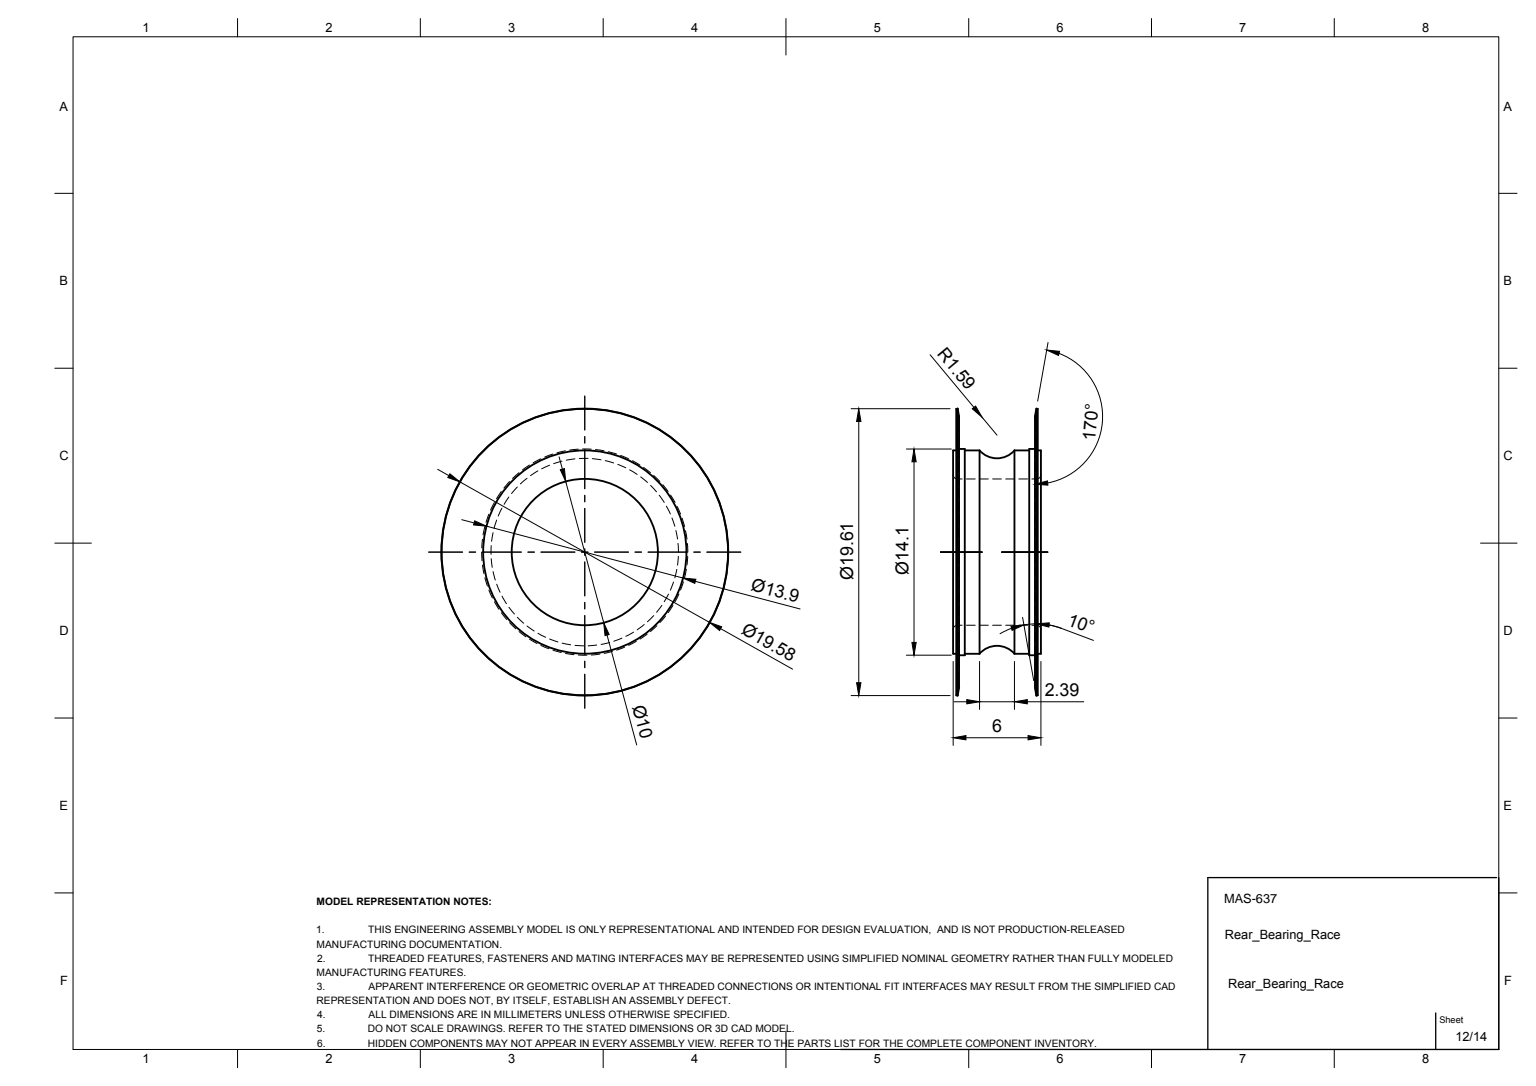
ISO-10303-21;
HEADER;
FILE_DESCRIPTION((''),'2;1');
FILE_NAME('Rear_Bearing_Race.step','2026-10-09T10:11:57-07:00',(''),(''),'','','');
FILE_SCHEMA (('AUTOMOTIVE_DESIGN { 1 0 10303 214 3 1 1 }'));
ENDSEC;
DATA;
#10=MECHANICAL_DESIGN_GEOMETRIC_PRESENTATION_REPRESENTATION('',(#144),#13510);
#105=SHAPE_REPRESENTATION_RELATIONSHIP('SRR','None',#13575,#120) ;
#120=ADVANCED_BREP_SHAPE_REPRESENTATION('',(#176),#13507) ;
#144=STYLED_ITEM('',(#13650),#176) ;
#176=MANIFOLD_SOLID_BREP('Body1',#7393) ;
#256=FACE_BOUND('',#1578,.T.) ;
#257=FACE_BOUND('',#1589,.T.) ;
#258=FACE_BOUND('',#1593,.T.) ;
#259=FACE_BOUND('',#1597,.T.) ;
#260=FACE_BOUND('',#1599,.T.) ;
#261=FACE_BOUND('',#1608,.T.) ;
#262=FACE_BOUND('',#1616,.T.) ;
#263=FACE_BOUND('',#1620,.T.) ;
#464=PLANE('',#8408) ;
#465=PLANE('',#8432) ;
#466=PLANE('',#8439) ;
#467=PLANE('',#8447) ;
#468=PLANE('',#8449) ;
#469=PLANE('',#8469) ;
#470=PLANE('',#8484) ;
#471=PLANE('',#8491) ;
#521=TOROIDAL_SURFACE('',#8404,7.1,0.15) ;
#522=TOROIDAL_SURFACE('',#8410,8.92946920772,0.45) ;
#523=TOROIDAL_SURFACE('',#8415,9.22752171828,0.349999999988) ;
#524=TOROIDAL_SURFACE('',#8424,9.22752171828,0.45) ;
#525=TOROIDAL_SURFACE('',#8429,8.92946920772,0.35) ;
#526=TOROIDAL_SURFACE('',#8434,7.1,0.05) ;
#527=TOROIDAL_SURFACE('',#8441,7.1,0.15) ;
#528=TOROIDAL_SURFACE('',#8451,8.92946920772,0.45) ;
#529=TOROIDAL_SURFACE('',#8454,5.3,0.3) ;
#530=TOROIDAL_SURFACE('',#8461,9.22752171828,0.349999999988) ;
#531=TOROIDAL_SURFACE('',#8464,5.3,0.3) ;
#532=TOROIDAL_SURFACE('',#8476,9.22752171828,0.45) ;
#533=TOROIDAL_SURFACE('',#8481,8.92946920772,0.35) ;
#534=TOROIDAL_SURFACE('',#8486,7.1,0.05) ;
#535=TOROIDAL_SURFACE('',#8495,8.,1.59) ;
#656=CYLINDRICAL_SURFACE('',#8437,7.05) ;
#657=CYLINDRICAL_SURFACE('',#8445,6.95) ;
#658=CYLINDRICAL_SURFACE('',#8459,5.) ;
#659=CYLINDRICAL_SURFACE('',#8473,6.95) ;
#660=CYLINDRICAL_SURFACE('',#8489,7.05) ;
#661=CYLINDRICAL_SURFACE('',#8493,6.95) ;
#662=CYLINDRICAL_SURFACE('',#8498,6.95) ;
#1059=FACE_OUTER_BOUND('',#1576,.T.) ;
#1060=FACE_OUTER_BOUND('',#1577,.T.) ;
#1061=FACE_OUTER_BOUND('',#1579,.T.) ;
#1062=FACE_OUTER_BOUND('',#1580,.T.) ;
#1063=FACE_OUTER_BOUND('',#1581,.T.) ;
#1064=FACE_OUTER_BOUND('',#1582,.T.) ;
#1065=FACE_OUTER_BOUND('',#1583,.T.) ;
#1066=FACE_OUTER_BOUND('',#1584,.T.) ;
#1067=FACE_OUTER_BOUND('',#1585,.T.) ;
#1068=FACE_OUTER_BOUND('',#1586,.T.) ;
#1069=FACE_OUTER_BOUND('',#1587,.T.) ;
#1070=FACE_OUTER_BOUND('',#1588,.T.) ;
#1071=FACE_OUTER_BOUND('',#1590,.T.) ;
#1072=FACE_OUTER_BOUND('',#1591,.T.) ;
#1073=FACE_OUTER_BOUND('',#1592,.T.) ;
#1074=FACE_OUTER_BOUND('',#1594,.T.) ;
#1075=FACE_OUTER_BOUND('',#1595,.T.) ;
#1076=FACE_OUTER_BOUND('',#1596,.T.) ;
#1077=FACE_OUTER_BOUND('',#1598,.T.) ;
#1078=FACE_OUTER_BOUND('',#1600,.T.) ;
#1079=FACE_OUTER_BOUND('',#1601,.T.) ;
#1080=FACE_OUTER_BOUND('',#1602,.T.) ;
#1081=FACE_OUTER_BOUND('',#1603,.T.) ;
#1082=FACE_OUTER_BOUND('',#1604,.T.) ;
#1083=FACE_OUTER_BOUND('',#1605,.T.) ;
#1084=FACE_OUTER_BOUND('',#1606,.T.) ;
#1085=FACE_OUTER_BOUND('',#1607,.T.) ;
#1086=FACE_OUTER_BOUND('',#1609,.T.) ;
#1087=FACE_OUTER_BOUND('',#1610,.T.) ;
#1088=FACE_OUTER_BOUND('',#1611,.T.) ;
#1089=FACE_OUTER_BOUND('',#1612,.T.) ;
#1090=FACE_OUTER_BOUND('',#1613,.T.) ;
#1091=FACE_OUTER_BOUND('',#1614,.T.) ;
#1092=FACE_OUTER_BOUND('',#1615,.T.) ;
#1093=FACE_OUTER_BOUND('',#1617,.T.) ;
#1094=FACE_OUTER_BOUND('',#1618,.T.) ;
#1095=FACE_OUTER_BOUND('',#1619,.T.) ;
#1096=FACE_OUTER_BOUND('',#1621,.T.) ;
#1097=FACE_OUTER_BOUND('',#1622,.T.) ;
#1098=FACE_OUTER_BOUND('',#1623,.T.) ;
#1576=EDGE_LOOP('',(#6656,#6657,#6658,#6659)) ;
#1577=EDGE_LOOP('',(#6660)) ;
#1578=EDGE_LOOP('',(#6661)) ;
#1579=EDGE_LOOP('',(#6662,#6663,#6664,#6665)) ;
#1580=EDGE_LOOP('',(#6666,#6667,#6668,#6669)) ;
#1581=EDGE_LOOP('',(#6670,#6671,#6672,#6673)) ;
#1582=EDGE_LOOP('',(#6674,#6675,#6676,#6677)) ;
#1583=EDGE_LOOP('',(#6678,#6679,#6680,#6681)) ;
#1584=EDGE_LOOP('',(#6682,#6683,#6684,#6685)) ;
#1585=EDGE_LOOP('',(#6686,#6687,#6688,#6689)) ;
#1586=EDGE_LOOP('',(#6690,#6691,#6692,#6693)) ;
#1587=EDGE_LOOP('',(#6694,#6695,#6696,#6697)) ;
#1588=EDGE_LOOP('',(#6698)) ;
#1589=EDGE_LOOP('',(#6699)) ;
#1590=EDGE_LOOP('',(#6700,#6701,#6702,#6703)) ;
#1591=EDGE_LOOP('',(#6704,#6705,#6706,#6707)) ;
#1592=EDGE_LOOP('',(#6708)) ;
#1593=EDGE_LOOP('',(#6709)) ;
#1594=EDGE_LOOP('',(#6710,#6711,#6712,#6713)) ;
#1595=EDGE_LOOP('',(#6714,#6715,#6716,#6717)) ;
#1596=EDGE_LOOP('',(#6718)) ;
#1597=EDGE_LOOP('',(#6719)) ;
#1598=EDGE_LOOP('',(#6720)) ;
#1599=EDGE_LOOP('',(#6721)) ;
#1600=EDGE_LOOP('',(#6722,#6723,#6724,#6725)) ;
#1601=EDGE_LOOP('',(#6726,#6727,#6728,#6729)) ;
#1602=EDGE_LOOP('',(#6730,#6731,#6732,#6733)) ;
#1603=EDGE_LOOP('',(#6734,#6735,#6736,#6737)) ;
#1604=EDGE_LOOP('',(#6738,#6739,#6740,#6741)) ;
#1605=EDGE_LOOP('',(#6742,#6743,#6744,#6745)) ;
#1606=EDGE_LOOP('',(#6746,#6747,#6748,#6749)) ;
#1607=EDGE_LOOP('',(#6750)) ;
#1608=EDGE_LOOP('',(#6751)) ;
#1609=EDGE_LOOP('',(#6752,#6753,#6754,#6755)) ;
#1610=EDGE_LOOP('',(#6756,#6757,#6758,#6759)) ;
#1611=EDGE_LOOP('',(#6760,#6761,#6762,#6763)) ;
#1612=EDGE_LOOP('',(#6764,#6765,#6766,#6767)) ;
#1613=EDGE_LOOP('',(#6768,#6769,#6770,#6771)) ;
#1614=EDGE_LOOP('',(#6772,#6773,#6774,#6775)) ;
#1615=EDGE_LOOP('',(#6776)) ;
#1616=EDGE_LOOP('',(#6777)) ;
#1617=EDGE_LOOP('',(#6778,#6779,#6780,#6781)) ;
#1618=EDGE_LOOP('',(#6782,#6783,#6784,#6785)) ;
#1619=EDGE_LOOP('',(#6786)) ;
#1620=EDGE_LOOP('',(#6787)) ;
#1621=EDGE_LOOP('',(#6788,#6789,#6790,#6791)) ;
#1622=EDGE_LOOP('',(#6792,#6793,#6794,#6795)) ;
#1623=EDGE_LOOP('',(#6796,#6797,#6798,#6799)) ;
#2119=LINE('',#13234,#2613) ;
#2120=LINE('',#13241,#2614) ;
#2121=LINE('',#13246,#2615) ;
#2122=LINE('',#13249,#2616) ;
#2123=LINE('',#13258,#2617) ;
#2124=LINE('',#13272,#2618) ;
#2125=LINE('',#13285,#2619) ;
#2126=LINE('',#13304,#2620) ;
#2127=LINE('',#13307,#2621) ;
#2128=LINE('',#13319,#2622) ;
#2129=LINE('',#13327,#2623) ;
#2130=LINE('',#13329,#2624) ;
#2131=LINE('',#13332,#2625) ;
#2132=LINE('',#13341,#2626) ;
#2133=LINE('',#13356,#2627) ;
#2134=LINE('',#13363,#2628) ;
#2135=LINE('',#13369,#2629) ;
#2613=VECTOR('',#10727,9.08337827221) ;
#2614=VECTOR('',#10736,9.28829858046) ;
#2615=VECTOR('',#10743,9.78979836642) ;
#2616=VECTOR('',#10746,9.30566339823) ;
#2617=VECTOR('',#10759,9.04917625788) ;
#2618=VECTOR('',#10778,7.05) ;
#2619=VECTOR('',#10795,6.95) ;
#2620=VECTOR('',#10822,9.08337827221) ;
#2621=VECTOR('',#10825,5.) ;
#2622=VECTOR('',#10842,9.28829858046) ;
#2623=VECTOR('',#10853,9.78979836642) ;
#2624=VECTOR('',#10856,6.95) ;
#2625=VECTOR('',#10859,9.30566339823) ;
#2626=VECTOR('',#10872,9.04917625788) ;
#2627=VECTOR('',#10893,7.05) ;
#2628=VECTOR('',#10902,6.95) ;
#2629=VECTOR('',#10911,6.95) ;
#3060=CIRCLE('',#8405,6.95) ;
#3061=CIRCLE('',#8406,0.15) ;
#3062=CIRCLE('',#8407,7.1) ;
#3063=CIRCLE('',#8409,8.92946920772) ;
#3064=CIRCLE('',#8411,0.45) ;
#3065=CIRCLE('',#8412,9.08337827221) ;
#3066=CIRCLE('',#8414,9.10781466811) ;
#3067=CIRCLE('',#8416,0.349999999988) ;
#3068=CIRCLE('',#8417,9.28829858046) ;
#3069=CIRCLE('',#8419,9.78979836642) ;
#3070=CIRCLE('',#8421,9.80716318419) ;
#3071=CIRCLE('',#8423,9.30566339823) ;
#3072=CIRCLE('',#8425,0.45) ;
#3073=CIRCLE('',#8426,9.07361265378) ;
#3074=CIRCLE('',#8428,9.04917625788) ;
#3075=CIRCLE('',#8430,0.35) ;
#3076=CIRCLE('',#8431,8.92946920772) ;
#3077=CIRCLE('',#8433,7.1) ;
#3078=CIRCLE('',#8435,0.05) ;
#3079=CIRCLE('',#8436,7.05) ;
#3080=CIRCLE('',#8438,7.05) ;
#3081=CIRCLE('',#8440,6.95) ;
#3082=CIRCLE('',#8442,7.1) ;
#3083=CIRCLE('',#8443,0.15) ;
#3084=CIRCLE('',#8444,6.95) ;
#3085=CIRCLE('',#8446,6.95) ;
#3086=CIRCLE('',#8448,8.92946920772) ;
#3087=CIRCLE('',#8450,5.3) ;
#3088=CIRCLE('',#8452,9.08337827221) ;
#3089=CIRCLE('',#8453,0.45) ;
#3090=CIRCLE('',#8455,0.3) ;
#3091=CIRCLE('',#8456,5.) ;
#3092=CIRCLE('',#8458,9.10781466811) ;
#3093=CIRCLE('',#8460,5.) ;
#3094=CIRCLE('',#8462,9.28829858046) ;
#3095=CIRCLE('',#8463,0.349999999988) ;
#3096=CIRCLE('',#8465,0.3) ;
#3097=CIRCLE('',#8466,5.3) ;
#3098=CIRCLE('',#8468,9.78979836642) ;
#3099=CIRCLE('',#8470,6.95) ;
#3100=CIRCLE('',#8472,9.80716318419) ;
#3101=CIRCLE('',#8475,9.30566339823) ;
#3102=CIRCLE('',#8477,9.07361265378) ;
#3103=CIRCLE('',#8478,0.45) ;
#3104=CIRCLE('',#8480,9.04917625788) ;
#3105=CIRCLE('',#8482,8.92946920772) ;
#3106=CIRCLE('',#8483,0.35) ;
#3107=CIRCLE('',#8485,7.1) ;
#3108=CIRCLE('',#8487,7.05) ;
#3109=CIRCLE('',#8488,0.05) ;
#3110=CIRCLE('',#8490,7.05) ;
#3111=CIRCLE('',#8492,6.95) ;
#3112=CIRCLE('',#8494,6.95) ;
#3113=CIRCLE('',#8496,6.95) ;
#3114=CIRCLE('',#8497,1.59) ;
#3726=VERTEX_POINT('',#13219) ;
#3727=VERTEX_POINT('',#13221) ;
#3728=VERTEX_POINT('',#13225) ;
#3729=VERTEX_POINT('',#13228) ;
#3730=VERTEX_POINT('',#13232) ;
#3731=VERTEX_POINT('',#13236) ;
#3732=VERTEX_POINT('',#13240) ;
#3733=VERTEX_POINT('',#13244) ;
#3734=VERTEX_POINT('',#13248) ;
#3735=VERTEX_POINT('',#13252) ;
#3736=VERTEX_POINT('',#13256) ;
#3737=VERTEX_POINT('',#13260) ;
#3738=VERTEX_POINT('',#13264) ;
#3739=VERTEX_POINT('',#13267) ;
#3740=VERTEX_POINT('',#13271) ;
#3741=VERTEX_POINT('',#13275) ;
#3742=VERTEX_POINT('',#13278) ;
#3743=VERTEX_POINT('',#13280) ;
#3744=VERTEX_POINT('',#13284) ;
#3745=VERTEX_POINT('',#13288) ;
#3746=VERTEX_POINT('',#13291) ;
#3747=VERTEX_POINT('',#13294) ;
#3748=VERTEX_POINT('',#13298) ;
#3749=VERTEX_POINT('',#13302) ;
#3750=VERTEX_POINT('',#13306) ;
#3751=VERTEX_POINT('',#13310) ;
#3752=VERTEX_POINT('',#13314) ;
#3753=VERTEX_POINT('',#13318) ;
#3754=VERTEX_POINT('',#13322) ;
#3755=VERTEX_POINT('',#13325) ;
#3756=VERTEX_POINT('',#13331) ;
#3757=VERTEX_POINT('',#13335) ;
#3758=VERTEX_POINT('',#13339) ;
#3759=VERTEX_POINT('',#13343) ;
#3760=VERTEX_POINT('',#13347) ;
#3761=VERTEX_POINT('',#13350) ;
#3762=VERTEX_POINT('',#13354) ;
#3763=VERTEX_POINT('',#13358) ;
#3764=VERTEX_POINT('',#13361) ;
#3765=VERTEX_POINT('',#13365) ;
#4715=EDGE_CURVE('',#3726,#3726,#3060,.T.) ;
#4716=EDGE_CURVE('',#3726,#3727,#3061,.T.) ;
#4717=EDGE_CURVE('',#3727,#3727,#3062,.T.) ;
#4718=EDGE_CURVE('',#3728,#3728,#3063,.T.) ;
#4719=EDGE_CURVE('',#3728,#3729,#3064,.T.) ;
#4720=EDGE_CURVE('',#3729,#3729,#3065,.T.) ;
#4721=EDGE_CURVE('',#3730,#3730,#3066,.F.) ;
#4722=EDGE_CURVE('',#3730,#3729,#2119,.T.) ;
#4723=EDGE_CURVE('',#3730,#3731,#3067,.T.) ;
#4724=EDGE_CURVE('',#3731,#3731,#3068,.T.) ;
#4725=EDGE_CURVE('',#3731,#3732,#2120,.T.) ;
#4726=EDGE_CURVE('',#3732,#3732,#3069,.T.) ;
#4727=EDGE_CURVE('',#3733,#3733,#3070,.F.) ;
#4728=EDGE_CURVE('',#3733,#3732,#2121,.T.) ;
#4729=EDGE_CURVE('',#3733,#3734,#2122,.T.) ;
#4730=EDGE_CURVE('',#3734,#3734,#3071,.T.) ;
#4731=EDGE_CURVE('',#3734,#3735,#3072,.T.) ;
#4732=EDGE_CURVE('',#3735,#3735,#3073,.T.) ;
#4733=EDGE_CURVE('',#3736,#3736,#3074,.F.) ;
#4734=EDGE_CURVE('',#3736,#3735,#2123,.T.) ;
#4735=EDGE_CURVE('',#3736,#3737,#3075,.T.) ;
#4736=EDGE_CURVE('',#3737,#3737,#3076,.T.) ;
#4737=EDGE_CURVE('',#3738,#3738,#3077,.T.) ;
#4738=EDGE_CURVE('',#3738,#3739,#3078,.T.) ;
#4739=EDGE_CURVE('',#3739,#3739,#3079,.T.) ;
#4740=EDGE_CURVE('',#3739,#3740,#2124,.T.) ;
#4741=EDGE_CURVE('',#3740,#3740,#3080,.T.) ;
#4742=EDGE_CURVE('',#3741,#3741,#3081,.T.) ;
#4743=EDGE_CURVE('',#3742,#3742,#3082,.T.) ;
#4744=EDGE_CURVE('',#3742,#3743,#3083,.T.) ;
#4745=EDGE_CURVE('',#3743,#3743,#3084,.T.) ;
#4746=EDGE_CURVE('',#3743,#3744,#2125,.T.) ;
#4747=EDGE_CURVE('',#3744,#3744,#3085,.T.) ;
#4748=EDGE_CURVE('',#3745,#3745,#3086,.T.) ;
#4749=EDGE_CURVE('',#3746,#3746,#3087,.T.) ;
#4750=EDGE_CURVE('',#3747,#3747,#3088,.T.) ;
#4751=EDGE_CURVE('',#3747,#3745,#3089,.T.) ;
#4752=EDGE_CURVE('',#3746,#3748,#3090,.T.) ;
#4753=EDGE_CURVE('',#3748,#3748,#3091,.T.) ;
#4754=EDGE_CURVE('',#3749,#3749,#3092,.T.) ;
#4755=EDGE_CURVE('',#3749,#3747,#2126,.T.) ;
#4756=EDGE_CURVE('',#3748,#3750,#2127,.T.) ;
#4757=EDGE_CURVE('',#3750,#3750,#3093,.T.) ;
#4758=EDGE_CURVE('',#3751,#3751,#3094,.T.) ;
#4759=EDGE_CURVE('',#3751,#3749,#3095,.T.) ;
#4760=EDGE_CURVE('',#3750,#3752,#3096,.T.) ;
#4761=EDGE_CURVE('',#3752,#3752,#3097,.T.) ;
#4762=EDGE_CURVE('',#3751,#3753,#2128,.T.) ;
#4763=EDGE_CURVE('',#3753,#3753,#3098,.F.) ;
#4764=EDGE_CURVE('',#3754,#3754,#3099,.T.) ;
#4765=EDGE_CURVE('',#3755,#3755,#3100,.T.) ;
#4766=EDGE_CURVE('',#3755,#3753,#2129,.T.) ;
#4767=EDGE_CURVE('',#3754,#3726,#2130,.T.) ;
#4768=EDGE_CURVE('',#3755,#3756,#2131,.T.) ;
#4769=EDGE_CURVE('',#3756,#3756,#3101,.F.) ;
#4770=EDGE_CURVE('',#3757,#3757,#3102,.T.) ;
#4771=EDGE_CURVE('',#3757,#3756,#3103,.T.) ;
#4772=EDGE_CURVE('',#3758,#3758,#3104,.T.) ;
#4773=EDGE_CURVE('',#3758,#3757,#2132,.T.) ;
#4774=EDGE_CURVE('',#3759,#3759,#3105,.T.) ;
#4775=EDGE_CURVE('',#3759,#3758,#3106,.T.) ;
#4776=EDGE_CURVE('',#3760,#3760,#3107,.T.) ;
#4777=EDGE_CURVE('',#3761,#3761,#3108,.T.) ;
#4778=EDGE_CURVE('',#3761,#3760,#3109,.T.) ;
#4779=EDGE_CURVE('',#3762,#3762,#3110,.T.) ;
#4780=EDGE_CURVE('',#3762,#3761,#2133,.T.) ;
#4781=EDGE_CURVE('',#3763,#3763,#3111,.T.) ;
#4782=EDGE_CURVE('',#3764,#3764,#3112,.T.) ;
#4783=EDGE_CURVE('',#3764,#3763,#2134,.T.) ;
#4784=EDGE_CURVE('',#3765,#3765,#3113,.T.) ;
#4785=EDGE_CURVE('',#3765,#3764,#3114,.T.) ;
#4786=EDGE_CURVE('',#3741,#3765,#2135,.T.) ;
#6656=ORIENTED_EDGE('',*,*,#4715,.F.) ;
#6657=ORIENTED_EDGE('',*,*,#4716,.T.) ;
#6658=ORIENTED_EDGE('',*,*,#4717,.T.) ;
#6659=ORIENTED_EDGE('',*,*,#4716,.F.) ;
#6660=ORIENTED_EDGE('',*,*,#4718,.T.) ;
#6661=ORIENTED_EDGE('',*,*,#4717,.F.) ;
#6662=ORIENTED_EDGE('',*,*,#4718,.F.) ;
#6663=ORIENTED_EDGE('',*,*,#4719,.T.) ;
#6664=ORIENTED_EDGE('',*,*,#4720,.T.) ;
#6665=ORIENTED_EDGE('',*,*,#4719,.F.) ;
#6666=ORIENTED_EDGE('',*,*,#4721,.T.) ;
#6667=ORIENTED_EDGE('',*,*,#4722,.T.) ;
#6668=ORIENTED_EDGE('',*,*,#4720,.F.) ;
#6669=ORIENTED_EDGE('',*,*,#4722,.F.) ;
#6670=ORIENTED_EDGE('',*,*,#4721,.F.) ;
#6671=ORIENTED_EDGE('',*,*,#4723,.T.) ;
#6672=ORIENTED_EDGE('',*,*,#4724,.T.) ;
#6673=ORIENTED_EDGE('',*,*,#4723,.F.) ;
#6674=ORIENTED_EDGE('',*,*,#4724,.F.) ;
#6675=ORIENTED_EDGE('',*,*,#4725,.T.) ;
#6676=ORIENTED_EDGE('',*,*,#4726,.T.) ;
#6677=ORIENTED_EDGE('',*,*,#4725,.F.) ;
#6678=ORIENTED_EDGE('',*,*,#4727,.T.) ;
#6679=ORIENTED_EDGE('',*,*,#4728,.T.) ;
#6680=ORIENTED_EDGE('',*,*,#4726,.F.) ;
#6681=ORIENTED_EDGE('',*,*,#4728,.F.) ;
#6682=ORIENTED_EDGE('',*,*,#4727,.F.) ;
#6683=ORIENTED_EDGE('',*,*,#4729,.T.) ;
#6684=ORIENTED_EDGE('',*,*,#4730,.T.) ;
#6685=ORIENTED_EDGE('',*,*,#4729,.F.) ;
#6686=ORIENTED_EDGE('',*,*,#4730,.F.) ;
#6687=ORIENTED_EDGE('',*,*,#4731,.T.) ;
#6688=ORIENTED_EDGE('',*,*,#4732,.T.) ;
#6689=ORIENTED_EDGE('',*,*,#4731,.F.) ;
#6690=ORIENTED_EDGE('',*,*,#4733,.T.) ;
#6691=ORIENTED_EDGE('',*,*,#4734,.T.) ;
#6692=ORIENTED_EDGE('',*,*,#4732,.F.) ;
#6693=ORIENTED_EDGE('',*,*,#4734,.F.) ;
#6694=ORIENTED_EDGE('',*,*,#4733,.F.) ;
#6695=ORIENTED_EDGE('',*,*,#4735,.T.) ;
#6696=ORIENTED_EDGE('',*,*,#4736,.T.) ;
#6697=ORIENTED_EDGE('',*,*,#4735,.F.) ;
#6698=ORIENTED_EDGE('',*,*,#4736,.F.) ;
#6699=ORIENTED_EDGE('',*,*,#4737,.T.) ;
#6700=ORIENTED_EDGE('',*,*,#4737,.F.) ;
#6701=ORIENTED_EDGE('',*,*,#4738,.T.) ;
#6702=ORIENTED_EDGE('',*,*,#4739,.T.) ;
#6703=ORIENTED_EDGE('',*,*,#4738,.F.) ;
#6704=ORIENTED_EDGE('',*,*,#4739,.F.) ;
#6705=ORIENTED_EDGE('',*,*,#4740,.T.) ;
#6706=ORIENTED_EDGE('',*,*,#4741,.T.) ;
#6707=ORIENTED_EDGE('',*,*,#4740,.F.) ;
#6708=ORIENTED_EDGE('',*,*,#4741,.F.) ;
#6709=ORIENTED_EDGE('',*,*,#4742,.T.) ;
#6710=ORIENTED_EDGE('',*,*,#4743,.F.) ;
#6711=ORIENTED_EDGE('',*,*,#4744,.T.) ;
#6712=ORIENTED_EDGE('',*,*,#4745,.T.) ;
#6713=ORIENTED_EDGE('',*,*,#4744,.F.) ;
#6714=ORIENTED_EDGE('',*,*,#4745,.F.) ;
#6715=ORIENTED_EDGE('',*,*,#4746,.T.) ;
#6716=ORIENTED_EDGE('',*,*,#4747,.T.) ;
#6717=ORIENTED_EDGE('',*,*,#4746,.F.) ;
#6718=ORIENTED_EDGE('',*,*,#4748,.F.) ;
#6719=ORIENTED_EDGE('',*,*,#4743,.T.) ;
#6720=ORIENTED_EDGE('',*,*,#4747,.F.) ;
#6721=ORIENTED_EDGE('',*,*,#4749,.T.) ;
#6722=ORIENTED_EDGE('',*,*,#4750,.F.) ;
#6723=ORIENTED_EDGE('',*,*,#4751,.T.) ;
#6724=ORIENTED_EDGE('',*,*,#4748,.T.) ;
#6725=ORIENTED_EDGE('',*,*,#4751,.F.) ;
#6726=ORIENTED_EDGE('',*,*,#4749,.F.) ;
#6727=ORIENTED_EDGE('',*,*,#4752,.T.) ;
#6728=ORIENTED_EDGE('',*,*,#4753,.T.) ;
#6729=ORIENTED_EDGE('',*,*,#4752,.F.) ;
#6730=ORIENTED_EDGE('',*,*,#4754,.F.) ;
#6731=ORIENTED_EDGE('',*,*,#4755,.T.) ;
#6732=ORIENTED_EDGE('',*,*,#4750,.T.) ;
#6733=ORIENTED_EDGE('',*,*,#4755,.F.) ;
#6734=ORIENTED_EDGE('',*,*,#4753,.F.) ;
#6735=ORIENTED_EDGE('',*,*,#4756,.T.) ;
#6736=ORIENTED_EDGE('',*,*,#4757,.T.) ;
#6737=ORIENTED_EDGE('',*,*,#4756,.F.) ;
#6738=ORIENTED_EDGE('',*,*,#4758,.F.) ;
#6739=ORIENTED_EDGE('',*,*,#4759,.T.) ;
#6740=ORIENTED_EDGE('',*,*,#4754,.T.) ;
#6741=ORIENTED_EDGE('',*,*,#4759,.F.) ;
#6742=ORIENTED_EDGE('',*,*,#4757,.F.) ;
#6743=ORIENTED_EDGE('',*,*,#4760,.T.) ;
#6744=ORIENTED_EDGE('',*,*,#4761,.T.) ;
#6745=ORIENTED_EDGE('',*,*,#4760,.F.) ;
#6746=ORIENTED_EDGE('',*,*,#4758,.T.) ;
#6747=ORIENTED_EDGE('',*,*,#4762,.T.) ;
#6748=ORIENTED_EDGE('',*,*,#4763,.F.) ;
#6749=ORIENTED_EDGE('',*,*,#4762,.F.) ;
#6750=ORIENTED_EDGE('',*,*,#4764,.T.) ;
#6751=ORIENTED_EDGE('',*,*,#4761,.F.) ;
#6752=ORIENTED_EDGE('',*,*,#4765,.F.) ;
#6753=ORIENTED_EDGE('',*,*,#4766,.T.) ;
#6754=ORIENTED_EDGE('',*,*,#4763,.T.) ;
#6755=ORIENTED_EDGE('',*,*,#4766,.F.) ;
#6756=ORIENTED_EDGE('',*,*,#4764,.F.) ;
#6757=ORIENTED_EDGE('',*,*,#4767,.T.) ;
#6758=ORIENTED_EDGE('',*,*,#4715,.T.) ;
#6759=ORIENTED_EDGE('',*,*,#4767,.F.) ;
#6760=ORIENTED_EDGE('',*,*,#4765,.T.) ;
#6761=ORIENTED_EDGE('',*,*,#4768,.T.) ;
#6762=ORIENTED_EDGE('',*,*,#4769,.F.) ;
#6763=ORIENTED_EDGE('',*,*,#4768,.F.) ;
#6764=ORIENTED_EDGE('',*,*,#4770,.F.) ;
#6765=ORIENTED_EDGE('',*,*,#4771,.T.) ;
#6766=ORIENTED_EDGE('',*,*,#4769,.T.) ;
#6767=ORIENTED_EDGE('',*,*,#4771,.F.) ;
#6768=ORIENTED_EDGE('',*,*,#4772,.F.) ;
#6769=ORIENTED_EDGE('',*,*,#4773,.T.) ;
#6770=ORIENTED_EDGE('',*,*,#4770,.T.) ;
#6771=ORIENTED_EDGE('',*,*,#4773,.F.) ;
#6772=ORIENTED_EDGE('',*,*,#4774,.F.) ;
#6773=ORIENTED_EDGE('',*,*,#4775,.T.) ;
#6774=ORIENTED_EDGE('',*,*,#4772,.T.) ;
#6775=ORIENTED_EDGE('',*,*,#4775,.F.) ;
#6776=ORIENTED_EDGE('',*,*,#4774,.T.) ;
#6777=ORIENTED_EDGE('',*,*,#4776,.F.) ;
#6778=ORIENTED_EDGE('',*,*,#4777,.F.) ;
#6779=ORIENTED_EDGE('',*,*,#4778,.T.) ;
#6780=ORIENTED_EDGE('',*,*,#4776,.T.) ;
#6781=ORIENTED_EDGE('',*,*,#4778,.F.) ;
#6782=ORIENTED_EDGE('',*,*,#4779,.F.) ;
#6783=ORIENTED_EDGE('',*,*,#4780,.T.) ;
#6784=ORIENTED_EDGE('',*,*,#4777,.T.) ;
#6785=ORIENTED_EDGE('',*,*,#4780,.F.) ;
#6786=ORIENTED_EDGE('',*,*,#4779,.T.) ;
#6787=ORIENTED_EDGE('',*,*,#4781,.F.) ;
#6788=ORIENTED_EDGE('',*,*,#4782,.F.) ;
#6789=ORIENTED_EDGE('',*,*,#4783,.T.) ;
#6790=ORIENTED_EDGE('',*,*,#4781,.T.) ;
#6791=ORIENTED_EDGE('',*,*,#4783,.F.) ;
#6792=ORIENTED_EDGE('',*,*,#4784,.F.) ;
#6793=ORIENTED_EDGE('',*,*,#4785,.T.) ;
#6794=ORIENTED_EDGE('',*,*,#4782,.T.) ;
#6795=ORIENTED_EDGE('',*,*,#4785,.F.) ;
#6796=ORIENTED_EDGE('',*,*,#4742,.F.) ;
#6797=ORIENTED_EDGE('',*,*,#4786,.T.) ;
#6798=ORIENTED_EDGE('',*,*,#4784,.T.) ;
#6799=ORIENTED_EDGE('',*,*,#4786,.F.) ;
#6906=CONICAL_SURFACE('',#8413,9.08337827221,1.2217304764) ;
#6907=CONICAL_SURFACE('',#8418,9.28829858046,1.3962634016) ;
#6908=CONICAL_SURFACE('',#8420,9.78979836642,0.174532925199) ;
#6909=CONICAL_SURFACE('',#8422,9.30566339823,1.3962634016) ;
#6910=CONICAL_SURFACE('',#8427,9.04917625788,1.2217304764) ;
#6911=CONICAL_SURFACE('',#8457,9.08337827221,1.2217304764) ;
#6912=CONICAL_SURFACE('',#8467,9.28829858046,1.3962634016) ;
#6913=CONICAL_SURFACE('',#8471,9.78979836642,0.1745329252) ;
#6914=CONICAL_SURFACE('',#8474,9.30566339823,1.3962634016) ;
#6915=CONICAL_SURFACE('',#8479,9.04917625788,1.2217304764) ;
#7309=ADVANCED_FACE('',(#1059),#521,.T.) ;
#7310=ADVANCED_FACE('',(#1060,#256),#464,.T.) ;
#7311=ADVANCED_FACE('',(#1061),#522,.T.) ;
#7312=ADVANCED_FACE('',(#1062),#6906,.T.) ;
#7313=ADVANCED_FACE('',(#1063),#523,.F.) ;
#7314=ADVANCED_FACE('',(#1064),#6907,.F.) ;
#7315=ADVANCED_FACE('',(#1065),#6908,.T.) ;
#7316=ADVANCED_FACE('',(#1066),#6909,.T.) ;
#7317=ADVANCED_FACE('',(#1067),#524,.T.) ;
#7318=ADVANCED_FACE('',(#1068),#6910,.F.) ;
#7319=ADVANCED_FACE('',(#1069),#525,.F.) ;
#7320=ADVANCED_FACE('',(#1070,#257),#465,.F.) ;
#7321=ADVANCED_FACE('',(#1071),#526,.F.) ;
#7322=ADVANCED_FACE('',(#1072),#656,.T.) ;
#7323=ADVANCED_FACE('',(#1073,#258),#466,.F.) ;
#7324=ADVANCED_FACE('',(#1074),#527,.T.) ;
#7325=ADVANCED_FACE('',(#1075),#657,.T.) ;
#7326=ADVANCED_FACE('',(#1076,#259),#467,.F.) ;
#7327=ADVANCED_FACE('',(#1077,#260),#468,.F.) ;
#7328=ADVANCED_FACE('',(#1078),#528,.T.) ;
#7329=ADVANCED_FACE('',(#1079),#529,.T.) ;
#7330=ADVANCED_FACE('',(#1080),#6911,.T.) ;
#7331=ADVANCED_FACE('',(#1081),#658,.F.) ;
#7332=ADVANCED_FACE('',(#1082),#530,.F.) ;
#7333=ADVANCED_FACE('',(#1083),#531,.T.) ;
#7334=ADVANCED_FACE('',(#1084),#6912,.F.) ;
#7335=ADVANCED_FACE('',(#1085,#261),#469,.T.) ;
#7336=ADVANCED_FACE('',(#1086),#6913,.T.) ;
#7337=ADVANCED_FACE('',(#1087),#659,.T.) ;
#7338=ADVANCED_FACE('',(#1088),#6914,.T.) ;
#7339=ADVANCED_FACE('',(#1089),#532,.T.) ;
#7340=ADVANCED_FACE('',(#1090),#6915,.F.) ;
#7341=ADVANCED_FACE('',(#1091),#533,.F.) ;
#7342=ADVANCED_FACE('',(#1092,#262),#470,.T.) ;
#7343=ADVANCED_FACE('',(#1093),#534,.F.) ;
#7344=ADVANCED_FACE('',(#1094),#660,.T.) ;
#7345=ADVANCED_FACE('',(#1095,#263),#471,.T.) ;
#7346=ADVANCED_FACE('',(#1096),#661,.T.) ;
#7347=ADVANCED_FACE('',(#1097),#535,.F.) ;
#7348=ADVANCED_FACE('',(#1098),#662,.T.) ;
#7393=CLOSED_SHELL('',(#7309,#7310,#7311,#7312,#7313,#7314,#7315,#7316,
#7317,#7318,#7319,#7320,#7321,#7322,#7323,#7324,#7325,#7326,#7327,#7328,
#7329,#7330,#7331,#7332,#7333,#7334,#7335,#7336,#7337,#7338,#7339,#7340,
#7341,#7342,#7343,#7344,#7345,#7346,#7347,#7348)) ;
#8403=AXIS2_PLACEMENT_3D('',#13217,#10703,#10704) ;
#8404=AXIS2_PLACEMENT_3D('',#13218,#10705,#10706) ;
#8405=AXIS2_PLACEMENT_3D('',#13220,#10707,#10708) ;
#8406=AXIS2_PLACEMENT_3D('',#13222,#10709,#10710) ;
#8407=AXIS2_PLACEMENT_3D('',#13223,#10711,#10712) ;
#8408=AXIS2_PLACEMENT_3D('',#13224,#10713,#10714) ;
#8409=AXIS2_PLACEMENT_3D('',#13226,#10715,#10716) ;
#8410=AXIS2_PLACEMENT_3D('',#13227,#10717,#10718) ;
#8411=AXIS2_PLACEMENT_3D('',#13229,#10719,#10720) ;
#8412=AXIS2_PLACEMENT_3D('',#13230,#10721,#10722) ;
#8413=AXIS2_PLACEMENT_3D('',#13231,#10723,#10724) ;
#8414=AXIS2_PLACEMENT_3D('',#13233,#10725,#10726) ;
#8415=AXIS2_PLACEMENT_3D('',#13235,#10728,#10729) ;
#8416=AXIS2_PLACEMENT_3D('',#13237,#10730,#10731) ;
#8417=AXIS2_PLACEMENT_3D('',#13238,#10732,#10733) ;
#8418=AXIS2_PLACEMENT_3D('',#13239,#10734,#10735) ;
#8419=AXIS2_PLACEMENT_3D('',#13242,#10737,#10738) ;
#8420=AXIS2_PLACEMENT_3D('',#13243,#10739,#10740) ;
#8421=AXIS2_PLACEMENT_3D('',#13245,#10741,#10742) ;
#8422=AXIS2_PLACEMENT_3D('',#13247,#10744,#10745) ;
#8423=AXIS2_PLACEMENT_3D('',#13250,#10747,#10748) ;
#8424=AXIS2_PLACEMENT_3D('',#13251,#10749,#10750) ;
#8425=AXIS2_PLACEMENT_3D('',#13253,#10751,#10752) ;
#8426=AXIS2_PLACEMENT_3D('',#13254,#10753,#10754) ;
#8427=AXIS2_PLACEMENT_3D('',#13255,#10755,#10756) ;
#8428=AXIS2_PLACEMENT_3D('',#13257,#10757,#10758) ;
#8429=AXIS2_PLACEMENT_3D('',#13259,#10760,#10761) ;
#8430=AXIS2_PLACEMENT_3D('',#13261,#10762,#10763) ;
#8431=AXIS2_PLACEMENT_3D('',#13262,#10764,#10765) ;
#8432=AXIS2_PLACEMENT_3D('',#13263,#10766,#10767) ;
#8433=AXIS2_PLACEMENT_3D('',#13265,#10768,#10769) ;
#8434=AXIS2_PLACEMENT_3D('',#13266,#10770,#10771) ;
#8435=AXIS2_PLACEMENT_3D('',#13268,#10772,#10773) ;
#8436=AXIS2_PLACEMENT_3D('',#13269,#10774,#10775) ;
#8437=AXIS2_PLACEMENT_3D('',#13270,#10776,#10777) ;
#8438=AXIS2_PLACEMENT_3D('',#13273,#10779,#10780) ;
#8439=AXIS2_PLACEMENT_3D('',#13274,#10781,#10782) ;
#8440=AXIS2_PLACEMENT_3D('',#13276,#10783,#10784) ;
#8441=AXIS2_PLACEMENT_3D('',#13277,#10785,#10786) ;
#8442=AXIS2_PLACEMENT_3D('',#13279,#10787,#10788) ;
#8443=AXIS2_PLACEMENT_3D('',#13281,#10789,#10790) ;
#8444=AXIS2_PLACEMENT_3D('',#13282,#10791,#10792) ;
#8445=AXIS2_PLACEMENT_3D('',#13283,#10793,#10794) ;
#8446=AXIS2_PLACEMENT_3D('',#13286,#10796,#10797) ;
#8447=AXIS2_PLACEMENT_3D('',#13287,#10798,#10799) ;
#8448=AXIS2_PLACEMENT_3D('',#13289,#10800,#10801) ;
#8449=AXIS2_PLACEMENT_3D('',#13290,#10802,#10803) ;
#8450=AXIS2_PLACEMENT_3D('',#13292,#10804,#10805) ;
#8451=AXIS2_PLACEMENT_3D('',#13293,#10806,#10807) ;
#8452=AXIS2_PLACEMENT_3D('',#13295,#10808,#10809) ;
#8453=AXIS2_PLACEMENT_3D('',#13296,#10810,#10811) ;
#8454=AXIS2_PLACEMENT_3D('',#13297,#10812,#10813) ;
#8455=AXIS2_PLACEMENT_3D('',#13299,#10814,#10815) ;
#8456=AXIS2_PLACEMENT_3D('',#13300,#10816,#10817) ;
#8457=AXIS2_PLACEMENT_3D('',#13301,#10818,#10819) ;
#8458=AXIS2_PLACEMENT_3D('',#13303,#10820,#10821) ;
#8459=AXIS2_PLACEMENT_3D('',#13305,#10823,#10824) ;
#8460=AXIS2_PLACEMENT_3D('',#13308,#10826,#10827) ;
#8461=AXIS2_PLACEMENT_3D('',#13309,#10828,#10829) ;
#8462=AXIS2_PLACEMENT_3D('',#13311,#10830,#10831) ;
#8463=AXIS2_PLACEMENT_3D('',#13312,#10832,#10833) ;
#8464=AXIS2_PLACEMENT_3D('',#13313,#10834,#10835) ;
#8465=AXIS2_PLACEMENT_3D('',#13315,#10836,#10837) ;
#8466=AXIS2_PLACEMENT_3D('',#13316,#10838,#10839) ;
#8467=AXIS2_PLACEMENT_3D('',#13317,#10840,#10841) ;
#8468=AXIS2_PLACEMENT_3D('',#13320,#10843,#10844) ;
#8469=AXIS2_PLACEMENT_3D('',#13321,#10845,#10846) ;
#8470=AXIS2_PLACEMENT_3D('',#13323,#10847,#10848) ;
#8471=AXIS2_PLACEMENT_3D('',#13324,#10849,#10850) ;
#8472=AXIS2_PLACEMENT_3D('',#13326,#10851,#10852) ;
#8473=AXIS2_PLACEMENT_3D('',#13328,#10854,#10855) ;
#8474=AXIS2_PLACEMENT_3D('',#13330,#10857,#10858) ;
#8475=AXIS2_PLACEMENT_3D('',#13333,#10860,#10861) ;
#8476=AXIS2_PLACEMENT_3D('',#13334,#10862,#10863) ;
#8477=AXIS2_PLACEMENT_3D('',#13336,#10864,#10865) ;
#8478=AXIS2_PLACEMENT_3D('',#13337,#10866,#10867) ;
#8479=AXIS2_PLACEMENT_3D('',#13338,#10868,#10869) ;
#8480=AXIS2_PLACEMENT_3D('',#13340,#10870,#10871) ;
#8481=AXIS2_PLACEMENT_3D('',#13342,#10873,#10874) ;
#8482=AXIS2_PLACEMENT_3D('',#13344,#10875,#10876) ;
#8483=AXIS2_PLACEMENT_3D('',#13345,#10877,#10878) ;
#8484=AXIS2_PLACEMENT_3D('',#13346,#10879,#10880) ;
#8485=AXIS2_PLACEMENT_3D('',#13348,#10881,#10882) ;
#8486=AXIS2_PLACEMENT_3D('',#13349,#10883,#10884) ;
#8487=AXIS2_PLACEMENT_3D('',#13351,#10885,#10886) ;
#8488=AXIS2_PLACEMENT_3D('',#13352,#10887,#10888) ;
#8489=AXIS2_PLACEMENT_3D('',#13353,#10889,#10890) ;
#8490=AXIS2_PLACEMENT_3D('',#13355,#10891,#10892) ;
#8491=AXIS2_PLACEMENT_3D('',#13357,#10894,#10895) ;
#8492=AXIS2_PLACEMENT_3D('',#13359,#10896,#10897) ;
#8493=AXIS2_PLACEMENT_3D('',#13360,#10898,#10899) ;
#8494=AXIS2_PLACEMENT_3D('',#13362,#10900,#10901) ;
#8495=AXIS2_PLACEMENT_3D('',#13364,#10903,#10904) ;
#8496=AXIS2_PLACEMENT_3D('',#13366,#10905,#10906) ;
#8497=AXIS2_PLACEMENT_3D('',#13367,#10907,#10908) ;
#8498=AXIS2_PLACEMENT_3D('',#13368,#10909,#10910) ;
#10703=DIRECTION('axis',(0.,0.,1.)) ;
#10704=DIRECTION('refdir',(1.,0.,0.)) ;
#10705=DIRECTION('center_axis',(0.,0.,-1.)) ;
#10706=DIRECTION('ref_axis',(0.877582561890372,-0.479425538604204,0.)) ;
#10707=DIRECTION('center_axis',(0.,0.,-1.)) ;
#10708=DIRECTION('ref_axis',(1.,0.,0.)) ;
#10709=DIRECTION('center_axis',(0.479425538604204,0.877582561890372,0.)) ;
#10710=DIRECTION('ref_axis',(-0.877582561890372,0.479425538604204,0.)) ;
#10711=DIRECTION('center_axis',(0.,0.,-1.)) ;
#10712=DIRECTION('ref_axis',(1.,0.,0.)) ;
#10713=DIRECTION('center_axis',(0.,0.,-1.)) ;
#10714=DIRECTION('ref_axis',(1.,0.,0.)) ;
#10715=DIRECTION('center_axis',(0.,0.,-1.)) ;
#10716=DIRECTION('ref_axis',(1.,0.,0.)) ;
#10717=DIRECTION('center_axis',(0.,0.,-1.)) ;
#10718=DIRECTION('ref_axis',(0.877582561890372,-0.479425538604204,0.)) ;
#10719=DIRECTION('center_axis',(0.479425538604204,0.877582561890372,0.)) ;
#10720=DIRECTION('ref_axis',(-0.877582561890372,0.479425538604204,0.)) ;
#10721=DIRECTION('center_axis',(0.,0.,-1.)) ;
#10722=DIRECTION('ref_axis',(1.,0.,0.)) ;
#10723=DIRECTION('center_axis',(0.,0.,1.)) ;
#10724=DIRECTION('ref_axis',(0.877582561890372,-0.479425538604204,0.)) ;
#10725=DIRECTION('center_axis',(0.,0.,1.)) ;
#10726=DIRECTION('ref_axis',(-1.,0.,0.)) ;
#10727=DIRECTION('',(0.824657857539967,-0.450512640843331,-0.342020143321939)) ;
#10728=DIRECTION('center_axis',(0.,0.,-1.)) ;
#10729=DIRECTION('ref_axis',(0.877582561890372,-0.479425538604204,0.)) ;
#10730=DIRECTION('center_axis',(-0.479425538604204,-0.877582561890372,0.)) ;
#10731=DIRECTION('ref_axis',(-0.877582561890372,0.479425538604204,0.)) ;
#10732=DIRECTION('center_axis',(0.,0.,-1.)) ;
#10733=DIRECTION('ref_axis',(1.,0.,0.)) ;
#10734=DIRECTION('center_axis',(0.,0.,-1.)) ;
#10735=DIRECTION('ref_axis',(0.877582561890372,-0.479425538604204,0.)) ;
#10736=DIRECTION('',(-0.864250110858646,0.472141987409852,-0.173648177662463)) ;
#10737=DIRECTION('center_axis',(0.,0.,-1.)) ;
#10738=DIRECTION('ref_axis',(1.,0.,0.)) ;
#10739=DIRECTION('center_axis',(0.,0.,1.)) ;
#10740=DIRECTION('ref_axis',(0.877582561890372,-0.479425538604204,0.)) ;
#10741=DIRECTION('center_axis',(0.,0.,1.)) ;
#10742=DIRECTION('ref_axis',(-1.,0.,0.)) ;
#10743=DIRECTION('',(0.152390612624165,-0.0832513711054022,-0.984807753012283)) ;
#10744=DIRECTION('center_axis',(0.,0.,-1.)) ;
#10745=DIRECTION('ref_axis',(0.877582561890372,-0.479425538604203,0.)) ;
#10746=DIRECTION('',(0.864250110858646,-0.472141987409851,0.173648177662463)) ;
#10747=DIRECTION('center_axis',(0.,0.,-1.)) ;
#10748=DIRECTION('ref_axis',(1.,0.,0.)) ;
#10749=DIRECTION('center_axis',(0.,0.,-1.)) ;
#10750=DIRECTION('ref_axis',(0.877582561890372,-0.479425538604204,0.)) ;
#10751=DIRECTION('center_axis',(0.479425538604204,0.877582561890372,0.)) ;
#10752=DIRECTION('ref_axis',(-0.877582561890372,0.479425538604204,0.)) ;
#10753=DIRECTION('center_axis',(0.,0.,-1.)) ;
#10754=DIRECTION('ref_axis',(1.,0.,0.)) ;
#10755=DIRECTION('center_axis',(0.,0.,1.)) ;
#10756=DIRECTION('ref_axis',(0.877582561890373,-0.479425538604203,0.)) ;
#10757=DIRECTION('center_axis',(0.,0.,1.)) ;
#10758=DIRECTION('ref_axis',(-1.,0.,0.)) ;
#10759=DIRECTION('',(-0.824657857539968,0.45051264084333,0.342020143321939)) ;
#10760=DIRECTION('center_axis',(0.,0.,-1.)) ;
#10761=DIRECTION('ref_axis',(0.877582561890372,-0.479425538604204,0.)) ;
#10762=DIRECTION('center_axis',(-0.479425538604204,-0.877582561890372,0.)) ;
#10763=DIRECTION('ref_axis',(-0.877582561890372,0.479425538604204,0.)) ;
#10764=DIRECTION('center_axis',(0.,0.,-1.)) ;
#10765=DIRECTION('ref_axis',(1.,0.,0.)) ;
#10766=DIRECTION('center_axis',(0.,0.,-1.)) ;
#10767=DIRECTION('ref_axis',(1.,0.,0.)) ;
#10768=DIRECTION('center_axis',(0.,0.,-1.)) ;
#10769=DIRECTION('ref_axis',(1.,0.,0.)) ;
#10770=DIRECTION('center_axis',(0.,0.,-1.)) ;
#10771=DIRECTION('ref_axis',(0.877582561890372,-0.479425538604204,0.)) ;
#10772=DIRECTION('center_axis',(-0.479425538604204,-0.877582561890372,0.)) ;
#10773=DIRECTION('ref_axis',(-0.877582561890372,0.479425538604204,0.)) ;
#10774=DIRECTION('center_axis',(0.,0.,-1.)) ;
#10775=DIRECTION('ref_axis',(1.,0.,0.)) ;
#10776=DIRECTION('center_axis',(0.,0.,-1.)) ;
#10777=DIRECTION('ref_axis',(0.877582561890372,-0.479425538604204,0.)) ;
#10778=DIRECTION('',(0.,0.,1.)) ;
#10779=DIRECTION('center_axis',(0.,0.,-1.)) ;
#10780=DIRECTION('ref_axis',(1.,0.,0.)) ;
#10781=DIRECTION('center_axis',(0.,0.,-1.)) ;
#10782=DIRECTION('ref_axis',(1.,0.,0.)) ;
#10783=DIRECTION('center_axis',(0.,0.,-1.)) ;
#10784=DIRECTION('ref_axis',(1.,0.,0.)) ;
#10785=DIRECTION('center_axis',(0.,0.,-1.)) ;
#10786=DIRECTION('ref_axis',(0.877582561890372,-0.479425538604204,0.)) ;
#10787=DIRECTION('center_axis',(0.,0.,-1.)) ;
#10788=DIRECTION('ref_axis',(1.,0.,0.)) ;
#10789=DIRECTION('center_axis',(0.479425538604204,0.877582561890372,0.)) ;
#10790=DIRECTION('ref_axis',(-0.877582561890372,0.479425538604204,0.)) ;
#10791=DIRECTION('center_axis',(0.,0.,-1.)) ;
#10792=DIRECTION('ref_axis',(1.,0.,0.)) ;
#10793=DIRECTION('center_axis',(0.,0.,-1.)) ;
#10794=DIRECTION('ref_axis',(0.877582561890373,-0.479425538604203,0.)) ;
#10795=DIRECTION('',(0.,0.,1.)) ;
#10796=DIRECTION('center_axis',(0.,0.,-1.)) ;
#10797=DIRECTION('ref_axis',(1.,0.,0.)) ;
#10798=DIRECTION('center_axis',(0.,0.,-1.)) ;
#10799=DIRECTION('ref_axis',(1.,0.,0.)) ;
#10800=DIRECTION('center_axis',(0.,0.,-1.)) ;
#10801=DIRECTION('ref_axis',(1.,0.,0.)) ;
#10802=DIRECTION('center_axis',(0.,0.,-1.)) ;
#10803=DIRECTION('ref_axis',(1.,0.,0.)) ;
#10804=DIRECTION('center_axis',(0.,0.,-1.)) ;
#10805=DIRECTION('ref_axis',(1.,0.,0.)) ;
#10806=DIRECTION('center_axis',(0.,0.,-1.)) ;
#10807=DIRECTION('ref_axis',(0.877582561890372,-0.479425538604204,0.)) ;
#10808=DIRECTION('center_axis',(0.,0.,-1.)) ;
#10809=DIRECTION('ref_axis',(1.,0.,0.)) ;
#10810=DIRECTION('center_axis',(0.479425538604204,0.877582561890372,0.)) ;
#10811=DIRECTION('ref_axis',(-0.877582561890372,0.479425538604204,0.)) ;
#10812=DIRECTION('center_axis',(0.,0.,-1.)) ;
#10813=DIRECTION('ref_axis',(0.877582561890372,-0.479425538604204,0.)) ;
#10814=DIRECTION('center_axis',(0.479425538604204,0.877582561890372,0.)) ;
#10815=DIRECTION('ref_axis',(-0.877582561890372,0.479425538604204,0.)) ;
#10816=DIRECTION('center_axis',(0.,0.,-1.)) ;
#10817=DIRECTION('ref_axis',(1.,0.,0.)) ;
#10818=DIRECTION('center_axis',(0.,0.,-1.)) ;
#10819=DIRECTION('ref_axis',(0.877582561890372,-0.479425538604204,0.)) ;
#10820=DIRECTION('center_axis',(0.,0.,-1.)) ;
#10821=DIRECTION('ref_axis',(1.,0.,0.)) ;
#10822=DIRECTION('',(0.824657857539967,-0.450512640843331,0.342020143321939)) ;
#10823=DIRECTION('center_axis',(0.,0.,-1.)) ;
#10824=DIRECTION('ref_axis',(0.877582561890372,-0.479425538604204,0.)) ;
#10825=DIRECTION('',(0.,0.,-1.)) ;
#10826=DIRECTION('center_axis',(0.,0.,-1.)) ;
#10827=DIRECTION('ref_axis',(1.,0.,0.)) ;
#10828=DIRECTION('center_axis',(0.,0.,-1.)) ;
#10829=DIRECTION('ref_axis',(0.877582561890372,-0.479425538604204,0.)) ;
#10830=DIRECTION('center_axis',(0.,0.,-1.)) ;
#10831=DIRECTION('ref_axis',(1.,0.,0.)) ;
#10832=DIRECTION('center_axis',(-0.479425538604204,-0.877582561890372,0.)) ;
#10833=DIRECTION('ref_axis',(-0.877582561890372,0.479425538604204,0.)) ;
#10834=DIRECTION('center_axis',(0.,0.,-1.)) ;
#10835=DIRECTION('ref_axis',(0.877582561890372,-0.479425538604204,0.)) ;
#10836=DIRECTION('center_axis',(0.479425538604204,0.877582561890372,0.)) ;
#10837=DIRECTION('ref_axis',(-0.877582561890372,0.479425538604204,0.)) ;
#10838=DIRECTION('center_axis',(0.,0.,-1.)) ;
#10839=DIRECTION('ref_axis',(1.,0.,0.)) ;
#10840=DIRECTION('center_axis',(0.,0.,1.)) ;
#10841=DIRECTION('ref_axis',(0.877582561890372,-0.479425538604204,0.)) ;
#10842=DIRECTION('',(-0.864250110858646,0.472141987409852,0.173648177662463)) ;
#10843=DIRECTION('center_axis',(0.,0.,1.)) ;
#10844=DIRECTION('ref_axis',(-1.,0.,0.)) ;
#10845=DIRECTION('center_axis',(0.,0.,-1.)) ;
#10846=DIRECTION('ref_axis',(1.,0.,0.)) ;
#10847=DIRECTION('center_axis',(0.,0.,-1.)) ;
#10848=DIRECTION('ref_axis',(1.,0.,0.)) ;
#10849=DIRECTION('center_axis',(0.,0.,-1.)) ;
#10850=DIRECTION('ref_axis',(0.877582561890372,-0.479425538604204,0.)) ;
#10851=DIRECTION('center_axis',(0.,0.,-1.)) ;
#10852=DIRECTION('ref_axis',(1.,0.,0.)) ;
#10853=DIRECTION('',(0.152390612625029,-0.0832513711058744,0.98480775301211)) ;
#10854=DIRECTION('center_axis',(0.,0.,-1.)) ;
#10855=DIRECTION('ref_axis',(0.877582561890373,-0.479425538604203,0.)) ;
#10856=DIRECTION('',(0.,0.,1.)) ;
#10857=DIRECTION('center_axis',(0.,0.,1.)) ;
#10858=DIRECTION('ref_axis',(0.877582561890372,-0.479425538604203,0.)) ;
#10859=DIRECTION('',(0.864250110858646,-0.472141987409851,-0.173648177662463)) ;
#10860=DIRECTION('center_axis',(0.,0.,1.)) ;
#10861=DIRECTION('ref_axis',(-1.,0.,0.)) ;
#10862=DIRECTION('center_axis',(0.,0.,-1.)) ;
#10863=DIRECTION('ref_axis',(0.877582561890372,-0.479425538604204,0.)) ;
#10864=DIRECTION('center_axis',(0.,0.,-1.)) ;
#10865=DIRECTION('ref_axis',(1.,0.,0.)) ;
#10866=DIRECTION('center_axis',(0.479425538604204,0.877582561890372,0.)) ;
#10867=DIRECTION('ref_axis',(-0.877582561890372,0.479425538604204,0.)) ;
#10868=DIRECTION('center_axis',(0.,0.,-1.)) ;
#10869=DIRECTION('ref_axis',(0.877582561890373,-0.479425538604203,0.)) ;
#10870=DIRECTION('center_axis',(0.,0.,-1.)) ;
#10871=DIRECTION('ref_axis',(1.,0.,0.)) ;
#10872=DIRECTION('',(-0.824657857539968,0.45051264084333,-0.342020143321939)) ;
#10873=DIRECTION('center_axis',(0.,0.,-1.)) ;
#10874=DIRECTION('ref_axis',(0.877582561890372,-0.479425538604204,0.)) ;
#10875=DIRECTION('center_axis',(0.,0.,-1.)) ;
#10876=DIRECTION('ref_axis',(1.,0.,0.)) ;
#10877=DIRECTION('center_axis',(-0.479425538604204,-0.877582561890372,0.)) ;
#10878=DIRECTION('ref_axis',(-0.877582561890372,0.479425538604204,0.)) ;
#10879=DIRECTION('center_axis',(0.,0.,-1.)) ;
#10880=DIRECTION('ref_axis',(1.,0.,0.)) ;
#10881=DIRECTION('center_axis',(0.,0.,-1.)) ;
#10882=DIRECTION('ref_axis',(1.,0.,0.)) ;
#10883=DIRECTION('center_axis',(0.,0.,-1.)) ;
#10884=DIRECTION('ref_axis',(0.877582561890372,-0.479425538604204,0.)) ;
#10885=DIRECTION('center_axis',(0.,0.,-1.)) ;
#10886=DIRECTION('ref_axis',(1.,0.,0.)) ;
#10887=DIRECTION('center_axis',(-0.479425538604204,-0.877582561890372,0.)) ;
#10888=DIRECTION('ref_axis',(-0.877582561890372,0.479425538604204,0.)) ;
#10889=DIRECTION('center_axis',(0.,0.,-1.)) ;
#10890=DIRECTION('ref_axis',(0.877582561890372,-0.479425538604204,0.)) ;
#10891=DIRECTION('center_axis',(0.,0.,-1.)) ;
#10892=DIRECTION('ref_axis',(1.,0.,0.)) ;
#10893=DIRECTION('',(0.,0.,1.)) ;
#10894=DIRECTION('center_axis',(0.,0.,-1.)) ;
#10895=DIRECTION('ref_axis',(1.,0.,0.)) ;
#10896=DIRECTION('center_axis',(0.,0.,-1.)) ;
#10897=DIRECTION('ref_axis',(1.,0.,0.)) ;
#10898=DIRECTION('center_axis',(0.,0.,-1.)) ;
#10899=DIRECTION('ref_axis',(0.877582561890373,-0.479425538604203,0.)) ;
#10900=DIRECTION('center_axis',(0.,0.,-1.)) ;
#10901=DIRECTION('ref_axis',(1.,0.,0.)) ;
#10902=DIRECTION('',(0.,0.,1.)) ;
#10903=DIRECTION('center_axis',(0.,0.,-1.)) ;
#10904=DIRECTION('ref_axis',(0.877582561890372,-0.479425538604204,0.)) ;
#10905=DIRECTION('center_axis',(0.,0.,-1.)) ;
#10906=DIRECTION('ref_axis',(1.,0.,0.)) ;
#10907=DIRECTION('center_axis',(-0.479425538604204,-0.877582561890372,0.)) ;
#10908=DIRECTION('ref_axis',(-0.877582561890372,0.479425538604204,0.)) ;
#10909=DIRECTION('center_axis',(0.,0.,-1.)) ;
#10910=DIRECTION('ref_axis',(0.877582561890373,-0.479425538604203,0.)) ;
#10911=DIRECTION('',(0.,0.,1.)) ;
#13217=CARTESIAN_POINT('',(0.,0.,0.)) ;
#13218=CARTESIAN_POINT('Origin',(0.,0.,109.4)) ;
#13219=CARTESIAN_POINT('',(-6.09919880514,3.3320074933,109.4)) ;
#13220=CARTESIAN_POINT('Origin',(0.,0.,109.4)) ;
#13221=CARTESIAN_POINT('',(-6.23083618942,3.40392132409,109.25)) ;
#13222=CARTESIAN_POINT('Origin',(-6.23083618942164,3.40392132408985,109.4)) ;
#13223=CARTESIAN_POINT('Origin',(0.,0.,109.25)) ;
#13224=CARTESIAN_POINT('Origin',(8.92946920772,0.,109.25)) ;
#13225=CARTESIAN_POINT('',(-7.83634646363211,4.28101558436081,109.25)) ;
#13226=CARTESIAN_POINT('Origin',(0.,0.,109.25)) ;
#13227=CARTESIAN_POINT('Origin',(0.,0.,109.7)) ;
#13228=CARTESIAN_POINT('',(-7.9714143747454,4.3548035205,109.277138321)) ;
#13229=CARTESIAN_POINT('Origin',(-7.83634646363211,4.28101558436082,109.7)) ;
#13230=CARTESIAN_POINT('Origin',(0.,0.,109.277138321)) ;
#13231=CARTESIAN_POINT('Origin',(0.,0.,109.277138321)) ;
#13232=CARTESIAN_POINT('',(-7.99285932967,4.36651895277,109.286032441)) ;
#13233=CARTESIAN_POINT('Origin',(0.,0.,109.286032441)) ;
#13234=CARTESIAN_POINT('',(-7.9714143747454,4.3548035205,109.277138321)) ;
#13235=CARTESIAN_POINT('Origin',(0.,0.,108.957140024)) ;
#13236=CARTESIAN_POINT('',(-8.15124886384,4.45304754965,109.301822738)) ;
#13237=CARTESIAN_POINT('Origin',(-8.09791214942721,4.42390956976838,108.957140024)) ;
#13238=CARTESIAN_POINT('Origin',(0.,0.,109.301822738)) ;
#13239=CARTESIAN_POINT('Origin',(0.,0.,109.301822738)) ;
#13240=CARTESIAN_POINT('',(-8.59135633079,4.69347935465,109.213394795)) ;
#13241=CARTESIAN_POINT('',(-8.15124886384279,4.4530475496537,109.301822738)) ;
#13242=CARTESIAN_POINT('Origin',(0.,0.,109.213394795)) ;
#13243=CARTESIAN_POINT('Origin',(0.,0.,109.213394795)) ;
#13244=CARTESIAN_POINT('',(-8.60659539201035,4.70180449173335,109.31187557001)) ;
#13245=CARTESIAN_POINT('Origin',(0.,0.,109.31187557)) ;
#13246=CARTESIAN_POINT('',(-8.59135633079305,4.69347935464747,109.213394795)) ;
#13247=CARTESIAN_POINT('Origin',(0.,0.,109.400303513)) ;
#13248=CARTESIAN_POINT('',(-8.16648792510815,4.46137268676584,109.400303513)) ;
#13249=CARTESIAN_POINT('',(-8.16648792510815,4.46137268676584,109.400303513)) ;
#13250=CARTESIAN_POINT('Origin',(0.,0.,109.400303513)) ;
#13251=CARTESIAN_POINT('Origin',(0.,0.,108.957140024)) ;
#13252=CARTESIAN_POINT('',(-7.96284423830515,4.35012163362439,109.380001703)) ;
#13253=CARTESIAN_POINT('Origin',(-8.09791214942721,4.42390956976838,108.957140024)) ;
#13254=CARTESIAN_POINT('Origin',(0.,0.,109.380001703)) ;
#13255=CARTESIAN_POINT('Origin',(0.,0.,109.371107583)) ;
#13256=CARTESIAN_POINT('',(-7.94139928338786,4.33840620135849,109.371107583)) ;
#13257=CARTESIAN_POINT('Origin',(0.,0.,109.371107583)) ;
#13258=CARTESIAN_POINT('',(-7.94139928338787,4.33840620135848,109.371107583)) ;
#13259=CARTESIAN_POINT('Origin',(0.,0.,109.7)) ;
#13260=CARTESIAN_POINT('',(-7.83634646363,4.28101558436,109.35)) ;
#13261=CARTESIAN_POINT('Origin',(-7.83634646363211,4.28101558436082,109.7)) ;
#13262=CARTESIAN_POINT('Origin',(0.,0.,109.35)) ;
#13263=CARTESIAN_POINT('Origin',(8.92946920772,0.,109.35)) ;
#13264=CARTESIAN_POINT('',(-6.23083618942164,3.40392132408985,109.35)) ;
#13265=CARTESIAN_POINT('Origin',(0.,0.,109.35)) ;
#13266=CARTESIAN_POINT('Origin',(0.,0.,109.4)) ;
#13267=CARTESIAN_POINT('',(-6.18695706132713,3.37995004715964,109.4)) ;
#13268=CARTESIAN_POINT('Origin',(-6.23083618942164,3.40392132408985,109.4)) ;
#13269=CARTESIAN_POINT('Origin',(0.,0.,109.4)) ;
#13270=CARTESIAN_POINT('Origin',(0.,0.,114.468682408)) ;
#13271=CARTESIAN_POINT('',(-6.18695706133,3.37995004716,109.8)) ;
#13272=CARTESIAN_POINT('',(-6.18695706132713,3.37995004715964,114.468682408)) ;
#13273=CARTESIAN_POINT('Origin',(0.,0.,109.8)) ;
#13274=CARTESIAN_POINT('Origin',(7.05,0.,109.8)) ;
#13275=CARTESIAN_POINT('',(-6.09919880514,3.3320074933,109.8)) ;
#13276=CARTESIAN_POINT('Origin',(0.,0.,109.8)) ;
#13277=CARTESIAN_POINT('Origin',(0.,0.,114.6)) ;
#13278=CARTESIAN_POINT('',(-6.23083618942164,3.40392132408985,114.75)) ;
#13279=CARTESIAN_POINT('Origin',(0.,0.,114.75)) ;
#13280=CARTESIAN_POINT('',(-6.09919880513809,3.33200749329922,114.6)) ;
#13281=CARTESIAN_POINT('Origin',(-6.23083618942164,3.40392132408985,114.6)) ;
#13282=CARTESIAN_POINT('Origin',(0.,0.,114.6)) ;
#13283=CARTESIAN_POINT('Origin',(0.,0.,112.)) ;
#13284=CARTESIAN_POINT('',(-6.09919880514,3.3320074933,115.)) ;
#13285=CARTESIAN_POINT('',(-6.09919880513809,3.33200749329921,112.)) ;
#13286=CARTESIAN_POINT('Origin',(0.,0.,115.)) ;
#13287=CARTESIAN_POINT('Origin',(8.92946920772,0.,114.75)) ;
#13288=CARTESIAN_POINT('',(-7.83634646363,4.28101558436,114.75)) ;
#13289=CARTESIAN_POINT('Origin',(0.,0.,114.75)) ;
#13290=CARTESIAN_POINT('Origin',(5.3,0.,115.)) ;
#13291=CARTESIAN_POINT('',(-4.65118757801897,2.54095535460228,115.)) ;
#13292=CARTESIAN_POINT('Origin',(0.,0.,115.)) ;
#13293=CARTESIAN_POINT('Origin',(0.,0.,114.3)) ;
#13294=CARTESIAN_POINT('',(-7.97141437475,4.3548035205,114.722861679)) ;
#13295=CARTESIAN_POINT('Origin',(0.,0.,114.722861679)) ;
#13296=CARTESIAN_POINT('Origin',(-7.83634646363211,4.28101558436082,114.3)) ;
#13297=CARTESIAN_POINT('Origin',(0.,0.,114.7)) ;
#13298=CARTESIAN_POINT('',(-4.38791280945186,2.39712769302102,114.7)) ;
#13299=CARTESIAN_POINT('Origin',(-4.65118757801897,2.54095535460228,114.7)) ;
#13300=CARTESIAN_POINT('Origin',(0.,0.,114.7)) ;
#13301=CARTESIAN_POINT('Origin',(0.,0.,114.722861679)) ;
#13302=CARTESIAN_POINT('',(-7.99285932945391,4.36651895265185,114.713967558346)) ;
#13303=CARTESIAN_POINT('Origin',(0.,0.,114.713967559)) ;
#13304=CARTESIAN_POINT('',(-7.9714143747454,4.35480352050001,114.722861679)) ;
#13305=CARTESIAN_POINT('Origin',(0.,0.,112.)) ;
#13306=CARTESIAN_POINT('',(-4.38791280945186,2.39712769302102,109.3)) ;
#13307=CARTESIAN_POINT('',(-4.38791280945186,2.39712769302102,112.)) ;
#13308=CARTESIAN_POINT('Origin',(0.,0.,109.3)) ;
#13309=CARTESIAN_POINT('Origin',(0.,0.,115.042859976)) ;
#13310=CARTESIAN_POINT('',(-8.1512488638428,4.45304754965369,114.698177262)) ;
#13311=CARTESIAN_POINT('Origin',(0.,0.,114.698177262)) ;
#13312=CARTESIAN_POINT('Origin',(-8.09791214942721,4.42390956976838,115.042859976)) ;
#13313=CARTESIAN_POINT('Origin',(0.,0.,109.3)) ;
#13314=CARTESIAN_POINT('',(-4.65118757801897,2.54095535460228,109.)) ;
#13315=CARTESIAN_POINT('Origin',(-4.65118757801897,2.54095535460228,109.3)) ;
#13316=CARTESIAN_POINT('Origin',(0.,0.,109.)) ;
#13317=CARTESIAN_POINT('Origin',(0.,0.,114.698177262)) ;
#13318=CARTESIAN_POINT('',(-8.59135633078075,4.69347935464074,114.786605205079)) ;
#13319=CARTESIAN_POINT('',(-8.15124886384279,4.4530475496537,114.698177262)) ;
#13320=CARTESIAN_POINT('Origin',(0.,0.,114.786605205)) ;
#13321=CARTESIAN_POINT('Origin',(5.3,0.,109.)) ;
#13322=CARTESIAN_POINT('',(-6.09919880514,3.3320074933,109.)) ;
#13323=CARTESIAN_POINT('Origin',(0.,0.,109.)) ;
#13324=CARTESIAN_POINT('Origin',(0.,0.,114.786605205)) ;
#13325=CARTESIAN_POINT('',(-8.60659539205,4.70180449176,114.68812443)) ;
#13326=CARTESIAN_POINT('Origin',(0.,0.,114.68812443)) ;
#13327=CARTESIAN_POINT('',(-8.59135633079304,4.69347935464747,114.786605205)) ;
#13328=CARTESIAN_POINT('Origin',(0.,0.,112.)) ;
#13329=CARTESIAN_POINT('',(-6.09919880513809,3.33200749329921,112.)) ;
#13330=CARTESIAN_POINT('Origin',(0.,0.,114.599696487)) ;
#13331=CARTESIAN_POINT('',(-8.16648792511,4.46137268677,114.599696487)) ;
#13332=CARTESIAN_POINT('',(-8.16648792510815,4.46137268676584,114.599696487)) ;
#13333=CARTESIAN_POINT('Origin',(0.,0.,114.599696487)) ;
#13334=CARTESIAN_POINT('Origin',(0.,0.,115.042859976)) ;
#13335=CARTESIAN_POINT('',(-7.96284423831,4.35012163363,114.619998297)) ;
#13336=CARTESIAN_POINT('Origin',(0.,0.,114.619998297)) ;
#13337=CARTESIAN_POINT('Origin',(-8.09791214942721,4.42390956976838,115.042859976)) ;
#13338=CARTESIAN_POINT('Origin',(0.,0.,114.628892417)) ;
#13339=CARTESIAN_POINT('',(-7.94139928339,4.33840620136,114.628892417)) ;
#13340=CARTESIAN_POINT('Origin',(0.,0.,114.628892417)) ;
#13341=CARTESIAN_POINT('',(-7.94139928338787,4.33840620135849,114.628892417)) ;
#13342=CARTESIAN_POINT('Origin',(0.,0.,114.3)) ;
#13343=CARTESIAN_POINT('',(-7.83634646363211,4.28101558436081,114.65)) ;
#13344=CARTESIAN_POINT('Origin',(0.,0.,114.65)) ;
#13345=CARTESIAN_POINT('Origin',(-7.83634646363211,4.28101558436082,114.3)) ;
#13346=CARTESIAN_POINT('Origin',(8.92946920772,0.,114.65)) ;
#13347=CARTESIAN_POINT('',(-6.23083618942,3.40392132409,114.65)) ;
#13348=CARTESIAN_POINT('Origin',(0.,0.,114.65)) ;
#13349=CARTESIAN_POINT('Origin',(0.,0.,114.6)) ;
#13350=CARTESIAN_POINT('',(-6.18695706133,3.37995004716,114.6)) ;
#13351=CARTESIAN_POINT('Origin',(0.,0.,114.6)) ;
#13352=CARTESIAN_POINT('Origin',(-6.23083618942164,3.40392132408985,114.6)) ;
#13353=CARTESIAN_POINT('Origin',(0.,0.,114.468682408)) ;
#13354=CARTESIAN_POINT('',(-6.18695706132713,3.37995004715963,114.2)) ;
#13355=CARTESIAN_POINT('Origin',(0.,0.,114.2)) ;
#13356=CARTESIAN_POINT('',(-6.18695706132713,3.37995004715964,114.468682408)) ;
#13357=CARTESIAN_POINT('Origin',(7.05,0.,114.2)) ;
#13358=CARTESIAN_POINT('',(-6.09919880513809,3.33200749329921,114.2)) ;
#13359=CARTESIAN_POINT('Origin',(0.,0.,114.2)) ;
#13360=CARTESIAN_POINT('Origin',(0.,0.,112.)) ;
#13361=CARTESIAN_POINT('',(-6.09919880513809,3.33200749329921,113.193984925)) ;
#13362=CARTESIAN_POINT('Origin',(0.,0.,113.193984925)) ;
#13363=CARTESIAN_POINT('',(-6.09919880513809,3.33200749329921,112.)) ;
#13364=CARTESIAN_POINT('Origin',(0.,0.,112.)) ;
#13365=CARTESIAN_POINT('',(-6.09919880514,3.3320074933,110.806015075)) ;
#13366=CARTESIAN_POINT('Origin',(0.,0.,110.806015075)) ;
#13367=CARTESIAN_POINT('Origin',(-7.02066049512298,3.83540430883363,112.)) ;
#13368=CARTESIAN_POINT('Origin',(0.,0.,112.)) ;
#13369=CARTESIAN_POINT('',(-6.09919880513809,3.33200749329921,112.)) ;
#13490=UNCERTAINTY_MEASURE_WITH_UNIT(LENGTH_MEASURE(0.01),#13511,
'DISTANCE_ACCURACY_VALUE',
'Maximum model space distance between geometric entities at asserted c
onnectivities') ;
#13493=UNCERTAINTY_MEASURE_WITH_UNIT(LENGTH_MEASURE(0.01),#13511,
'DISTANCE_ACCURACY_VALUE',
'Maximum model space distance between geometric entities at asserted c
onnectivities') ;
#13507=(
GEOMETRIC_REPRESENTATION_CONTEXT(3)
GLOBAL_UNCERTAINTY_ASSIGNED_CONTEXT((#13490))
GLOBAL_UNIT_ASSIGNED_CONTEXT((#13511,#13513,#13514))
REPRESENTATION_CONTEXT('','3D')
) ;
#13510=(
GEOMETRIC_REPRESENTATION_CONTEXT(3)
GLOBAL_UNCERTAINTY_ASSIGNED_CONTEXT((#13493))
GLOBAL_UNIT_ASSIGNED_CONTEXT((#13511,#13513,#13514))
REPRESENTATION_CONTEXT('','3D')
) ;
#13511=(
LENGTH_UNIT()
NAMED_UNIT(*)
SI_UNIT(.MILLI.,.METRE.)
) ;
#13513=(
NAMED_UNIT(*)
PLANE_ANGLE_UNIT()
SI_UNIT($,.RADIAN.)
) ;
#13514=(
NAMED_UNIT(*)
SI_UNIT($,.STERADIAN.)
SOLID_ANGLE_UNIT()
) ;
#13528=SHAPE_DEFINITION_REPRESENTATION(#13544,#13575) ;
#13544=PRODUCT_DEFINITION_SHAPE('',$,#13592) ;
#13575=SHAPE_REPRESENTATION('',(#8403),#13507) ;
#13578=PRODUCT_DEFINITION_CONTEXT('part definition',#13628,'design') ;
#13592=PRODUCT_DEFINITION('Rear_Bearing_Race','Rear_Bearing_Race',#13608,
#13578) ;
#13608=PRODUCT_DEFINITION_FORMATION('',$,#13643) ;
#13628=APPLICATION_CONTEXT(
'Core Data for Automotive Mechanical Design Process') ;
#13629=PRODUCT_CONTEXT('part definition',#13628,'mechanical') ;
#13643=PRODUCT('Rear_Bearing_Race','Rear_Bearing_Race',$,(#13629)) ;
#13650=PRESENTATION_STYLE_ASSIGNMENT((#13655)) ;
#13655=SURFACE_STYLE_USAGE(.BOTH.,#13660) ;
#13660=SURFACE_SIDE_STYLE('',(#13665)) ;
#13665=SURFACE_STYLE_FILL_AREA(#13670) ;
#13670=FILL_AREA_STYLE('Opaque(144,144,144)',(#13675)) ;
#13675=FILL_AREA_STYLE_COLOUR('Opaque(144,144,144)',#13680) ;
#13680=COLOUR_RGB('Opaque(144,144,144)', 0.40784314, 0.44705882, 0.49803922) ;
ENDSEC;
END-ISO-10303-21;
